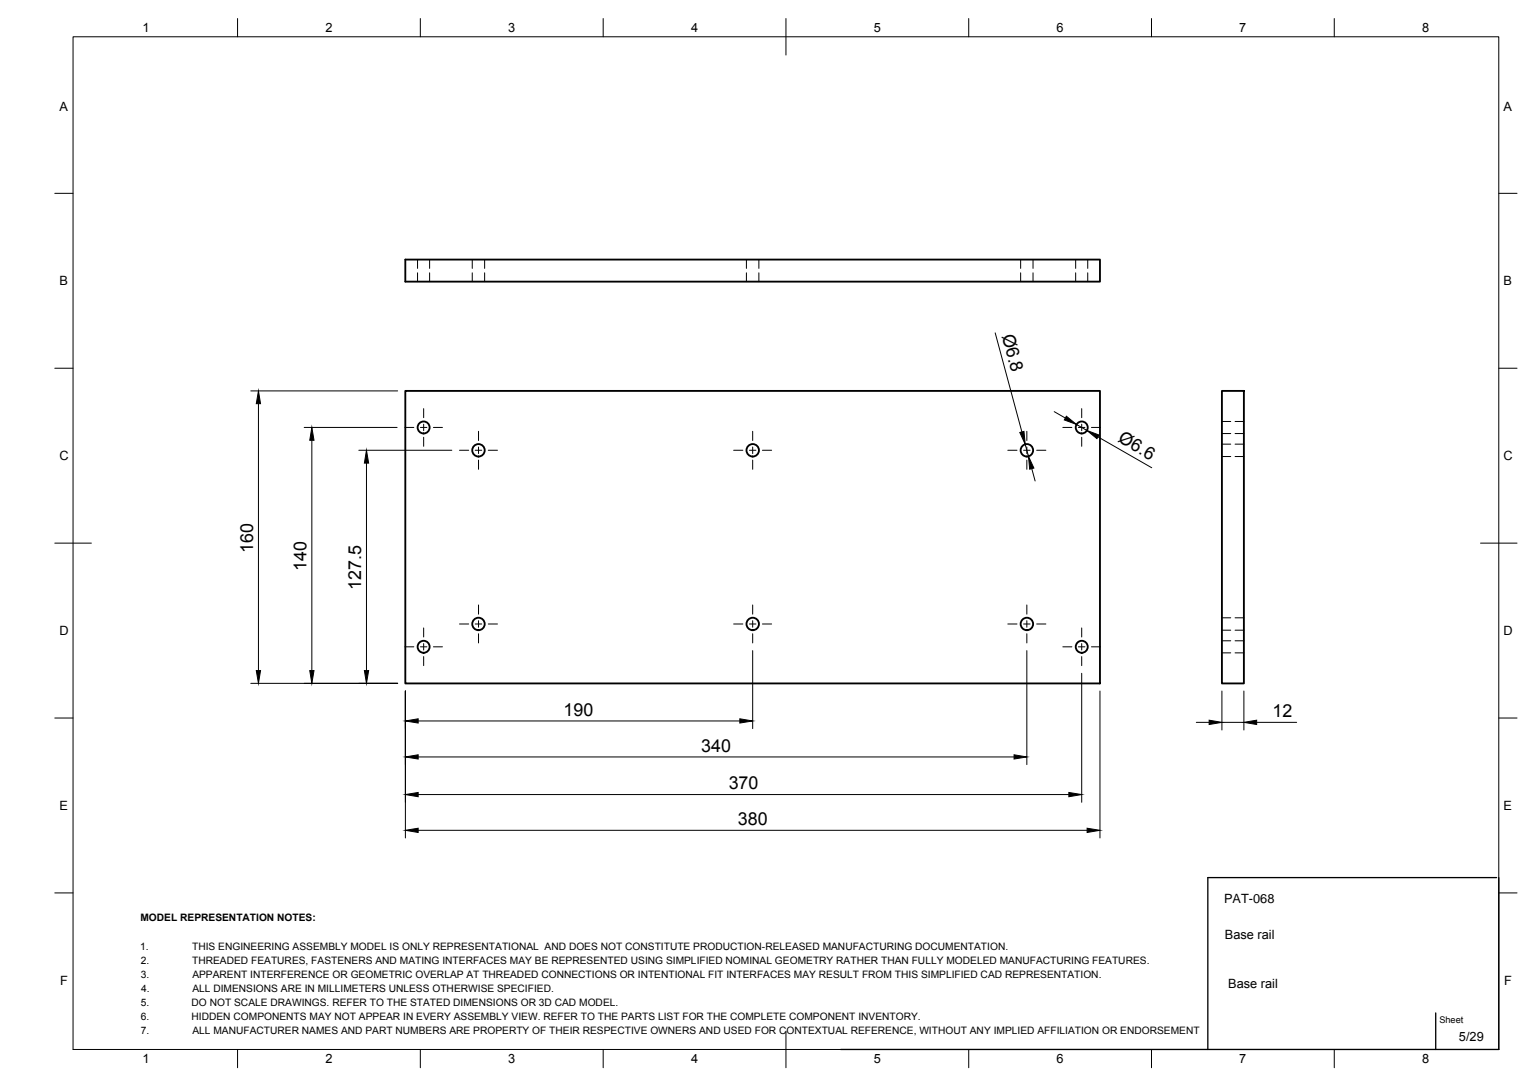
ISO-10303-21;
HEADER;
/* Generated by software containing ST-Developer
 * from STEP Tools, Inc. (www.steptools.com) 
 */

FILE_DESCRIPTION(
/* description */ ('Line shaft on three pillow blocks'),
/* implementation_level */ '2;1');

FILE_NAME(
/* name */ 'Base rail.step',
/* time_stamp */ '2026-10-27T10:49:19-07:00',
/* author */ (''),
/* organization */ (''),
/* preprocessor_version */ 'ST-DEVELOPER v20.2',
/* originating_system */ 'Autodesk Translation Framework v15.17.0.0',
/* authorisation */ '');

FILE_SCHEMA (('AUTOMOTIVE_DESIGN { 1 0 10303 214 3 1 1 }'));
ENDSEC;

DATA;
#10=MECHANICAL_DESIGN_GEOMETRIC_PRESENTATION_REPRESENTATION('',(#338),#8377);
#284=SHAPE_REPRESENTATION_RELATIONSHIP('SRR','None',#8499,#311);
#311=ADVANCED_BREP_SHAPE_REPRESENTATION('',(#366),#8348);
#338=STYLED_ITEM('',(#8697),#366);
#366=MANIFOLD_SOLID_BREP('Body1',#4324);
#391=FACE_BOUND('',#921,.T.);
#392=FACE_BOUND('',#922,.T.);
#393=FACE_BOUND('',#923,.T.);
#394=FACE_BOUND('',#924,.T.);
#395=FACE_BOUND('',#925,.T.);
#396=FACE_BOUND('',#926,.T.);
#397=FACE_BOUND('',#927,.T.);
#398=FACE_BOUND('',#928,.T.);
#399=FACE_BOUND('',#929,.T.);
#400=FACE_BOUND('',#930,.T.);
#401=FACE_BOUND('',#932,.T.);
#402=FACE_BOUND('',#933,.T.);
#403=FACE_BOUND('',#934,.T.);
#404=FACE_BOUND('',#935,.T.);
#405=FACE_BOUND('',#936,.T.);
#406=FACE_BOUND('',#937,.T.);
#407=FACE_BOUND('',#938,.T.);
#408=FACE_BOUND('',#939,.T.);
#409=FACE_BOUND('',#940,.T.);
#410=FACE_BOUND('',#941,.T.);
#488=PLANE('',#4686);
#489=PLANE('',#4687);
#490=PLANE('',#4688);
#491=PLANE('',#4689);
#492=PLANE('',#4690);
#493=PLANE('',#4691);
#654=FACE_OUTER_BOUND('',#906,.T.);
#655=FACE_OUTER_BOUND('',#907,.T.);
#656=FACE_OUTER_BOUND('',#908,.T.);
#657=FACE_OUTER_BOUND('',#909,.T.);
#658=FACE_OUTER_BOUND('',#910,.T.);
#659=FACE_OUTER_BOUND('',#911,.T.);
#660=FACE_OUTER_BOUND('',#912,.T.);
#661=FACE_OUTER_BOUND('',#913,.T.);
#662=FACE_OUTER_BOUND('',#914,.T.);
#663=FACE_OUTER_BOUND('',#915,.T.);
#664=FACE_OUTER_BOUND('',#916,.T.);
#665=FACE_OUTER_BOUND('',#917,.T.);
#666=FACE_OUTER_BOUND('',#918,.T.);
#667=FACE_OUTER_BOUND('',#919,.T.);
#668=FACE_OUTER_BOUND('',#920,.T.);
#669=FACE_OUTER_BOUND('',#931,.T.);
#906=EDGE_LOOP('',(#2949,#2950,#2951,#2952));
#907=EDGE_LOOP('',(#2953,#2954,#2955,#2956));
#908=EDGE_LOOP('',(#2957,#2958,#2959,#2960));
#909=EDGE_LOOP('',(#2961,#2962,#2963,#2964));
#910=EDGE_LOOP('',(#2965,#2966,#2967,#2968));
#911=EDGE_LOOP('',(#2969,#2970,#2971,#2972));
#912=EDGE_LOOP('',(#2973,#2974,#2975,#2976));
#913=EDGE_LOOP('',(#2977,#2978,#2979,#2980));
#914=EDGE_LOOP('',(#2981,#2982,#2983,#2984));
#915=EDGE_LOOP('',(#2985,#2986,#2987,#2988));
#916=EDGE_LOOP('',(#2989,#2990,#2991,#2992));
#917=EDGE_LOOP('',(#2993,#2994,#2995,#2996));
#918=EDGE_LOOP('',(#2997,#2998,#2999,#3000));
#919=EDGE_LOOP('',(#3001,#3002,#3003,#3004));
#920=EDGE_LOOP('',(#3005,#3006,#3007,#3008));
#921=EDGE_LOOP('',(#3009));
#922=EDGE_LOOP('',(#3010));
#923=EDGE_LOOP('',(#3011));
#924=EDGE_LOOP('',(#3012));
#925=EDGE_LOOP('',(#3013));
#926=EDGE_LOOP('',(#3014));
#927=EDGE_LOOP('',(#3015));
#928=EDGE_LOOP('',(#3016));
#929=EDGE_LOOP('',(#3017));
#930=EDGE_LOOP('',(#3018));
#931=EDGE_LOOP('',(#3019,#3020,#3021,#3022));
#932=EDGE_LOOP('',(#3023));
#933=EDGE_LOOP('',(#3024));
#934=EDGE_LOOP('',(#3025));
#935=EDGE_LOOP('',(#3026));
#936=EDGE_LOOP('',(#3027));
#937=EDGE_LOOP('',(#3028));
#938=EDGE_LOOP('',(#3029));
#939=EDGE_LOOP('',(#3030));
#940=EDGE_LOOP('',(#3031));
#941=EDGE_LOOP('',(#3032));
#1255=LINE('',#6472,#1582);
#1256=LINE('',#6478,#1583);
#1257=LINE('',#6484,#1584);
#1258=LINE('',#6490,#1585);
#1259=LINE('',#6496,#1586);
#1260=LINE('',#6502,#1587);
#1261=LINE('',#6508,#1588);
#1262=LINE('',#6514,#1589);
#1263=LINE('',#6520,#1590);
#1264=LINE('',#6526,#1591);
#1265=LINE('',#6531,#1592);
#1266=LINE('',#6533,#1593);
#1267=LINE('',#6535,#1594);
#1268=LINE('',#6536,#1595);
#1269=LINE('',#6539,#1596);
#1270=LINE('',#6541,#1597);
#1271=LINE('',#6542,#1598);
#1272=LINE('',#6545,#1599);
#1273=LINE('',#6547,#1600);
#1274=LINE('',#6548,#1601);
#1275=LINE('',#6550,#1602);
#1276=LINE('',#6551,#1603);
#1582=VECTOR('',#5158,0.33);
#1583=VECTOR('',#5165,0.33);
#1584=VECTOR('',#5172,0.33);
#1585=VECTOR('',#5179,0.33);
#1586=VECTOR('',#5186,0.34);
#1587=VECTOR('',#5193,0.34);
#1588=VECTOR('',#5200,0.34);
#1589=VECTOR('',#5207,0.34);
#1590=VECTOR('',#5214,0.34);
#1591=VECTOR('',#5221,0.34);
#1592=VECTOR('',#5226,1.);
#1593=VECTOR('',#5227,1.);
#1594=VECTOR('',#5228,1.);
#1595=VECTOR('',#5229,1.);
#1596=VECTOR('',#5232,1.);
#1597=VECTOR('',#5233,1.);
#1598=VECTOR('',#5234,1.);
#1599=VECTOR('',#5237,1.);
#1600=VECTOR('',#5238,1.);
#1601=VECTOR('',#5239,1.);
#1602=VECTOR('',#5242,1.);
#1603=VECTOR('',#5243,1.);
#1909=CIRCLE('',#4657,0.33);
#1910=CIRCLE('',#4658,0.33);
#1911=CIRCLE('',#4660,0.33);
#1912=CIRCLE('',#4661,0.33);
#1913=CIRCLE('',#4663,0.33);
#1914=CIRCLE('',#4664,0.33);
#1915=CIRCLE('',#4666,0.33);
#1916=CIRCLE('',#4667,0.33);
#1917=CIRCLE('',#4669,0.34);
#1918=CIRCLE('',#4670,0.34);
#1919=CIRCLE('',#4672,0.34);
#1920=CIRCLE('',#4673,0.34);
#1921=CIRCLE('',#4675,0.34);
#1922=CIRCLE('',#4676,0.34);
#1923=CIRCLE('',#4678,0.34);
#1924=CIRCLE('',#4679,0.34);
#1925=CIRCLE('',#4681,0.34);
#1926=CIRCLE('',#4682,0.34);
#1927=CIRCLE('',#4684,0.34);
#1928=CIRCLE('',#4685,0.34);
#2068=VERTEX_POINT('',#6469);
#2069=VERTEX_POINT('',#6471);
#2070=VERTEX_POINT('',#6475);
#2071=VERTEX_POINT('',#6477);
#2072=VERTEX_POINT('',#6481);
#2073=VERTEX_POINT('',#6483);
#2074=VERTEX_POINT('',#6487);
#2075=VERTEX_POINT('',#6489);
#2076=VERTEX_POINT('',#6493);
#2077=VERTEX_POINT('',#6495);
#2078=VERTEX_POINT('',#6499);
#2079=VERTEX_POINT('',#6501);
#2080=VERTEX_POINT('',#6505);
#2081=VERTEX_POINT('',#6507);
#2082=VERTEX_POINT('',#6511);
#2083=VERTEX_POINT('',#6513);
#2084=VERTEX_POINT('',#6517);
#2085=VERTEX_POINT('',#6519);
#2086=VERTEX_POINT('',#6523);
#2087=VERTEX_POINT('',#6525);
#2088=VERTEX_POINT('',#6529);
#2089=VERTEX_POINT('',#6530);
#2090=VERTEX_POINT('',#6532);
#2091=VERTEX_POINT('',#6534);
#2092=VERTEX_POINT('',#6538);
#2093=VERTEX_POINT('',#6540);
#2094=VERTEX_POINT('',#6544);
#2095=VERTEX_POINT('',#6546);
#2423=EDGE_CURVE('',#2068,#2068,#1909,.T.);
#2424=EDGE_CURVE('',#2068,#2069,#1255,.T.);
#2425=EDGE_CURVE('',#2069,#2069,#1910,.T.);
#2426=EDGE_CURVE('',#2070,#2070,#1911,.T.);
#2427=EDGE_CURVE('',#2070,#2071,#1256,.T.);
#2428=EDGE_CURVE('',#2071,#2071,#1912,.T.);
#2429=EDGE_CURVE('',#2072,#2072,#1913,.T.);
#2430=EDGE_CURVE('',#2072,#2073,#1257,.T.);
#2431=EDGE_CURVE('',#2073,#2073,#1914,.T.);
#2432=EDGE_CURVE('',#2074,#2074,#1915,.T.);
#2433=EDGE_CURVE('',#2074,#2075,#1258,.T.);
#2434=EDGE_CURVE('',#2075,#2075,#1916,.T.);
#2435=EDGE_CURVE('',#2076,#2076,#1917,.T.);
#2436=EDGE_CURVE('',#2076,#2077,#1259,.T.);
#2437=EDGE_CURVE('',#2077,#2077,#1918,.T.);
#2438=EDGE_CURVE('',#2078,#2078,#1919,.T.);
#2439=EDGE_CURVE('',#2078,#2079,#1260,.T.);
#2440=EDGE_CURVE('',#2079,#2079,#1920,.T.);
#2441=EDGE_CURVE('',#2080,#2080,#1921,.T.);
#2442=EDGE_CURVE('',#2080,#2081,#1261,.T.);
#2443=EDGE_CURVE('',#2081,#2081,#1922,.T.);
#2444=EDGE_CURVE('',#2082,#2082,#1923,.T.);
#2445=EDGE_CURVE('',#2082,#2083,#1262,.T.);
#2446=EDGE_CURVE('',#2083,#2083,#1924,.T.);
#2447=EDGE_CURVE('',#2084,#2084,#1925,.T.);
#2448=EDGE_CURVE('',#2084,#2085,#1263,.T.);
#2449=EDGE_CURVE('',#2085,#2085,#1926,.T.);
#2450=EDGE_CURVE('',#2086,#2086,#1927,.T.);
#2451=EDGE_CURVE('',#2086,#2087,#1264,.T.);
#2452=EDGE_CURVE('',#2087,#2087,#1928,.T.);
#2453=EDGE_CURVE('',#2088,#2089,#1265,.T.);
#2454=EDGE_CURVE('',#2089,#2090,#1266,.T.);
#2455=EDGE_CURVE('',#2091,#2090,#1267,.T.);
#2456=EDGE_CURVE('',#2088,#2091,#1268,.T.);
#2457=EDGE_CURVE('',#2092,#2088,#1269,.T.);
#2458=EDGE_CURVE('',#2093,#2091,#1270,.T.);
#2459=EDGE_CURVE('',#2092,#2093,#1271,.T.);
#2460=EDGE_CURVE('',#2094,#2092,#1272,.T.);
#2461=EDGE_CURVE('',#2095,#2093,#1273,.T.);
#2462=EDGE_CURVE('',#2094,#2095,#1274,.T.);
#2463=EDGE_CURVE('',#2089,#2094,#1275,.T.);
#2464=EDGE_CURVE('',#2090,#2095,#1276,.T.);
#2949=ORIENTED_EDGE('',*,*,#2423,.F.);
#2950=ORIENTED_EDGE('',*,*,#2424,.T.);
#2951=ORIENTED_EDGE('',*,*,#2425,.F.);
#2952=ORIENTED_EDGE('',*,*,#2424,.F.);
#2953=ORIENTED_EDGE('',*,*,#2426,.F.);
#2954=ORIENTED_EDGE('',*,*,#2427,.T.);
#2955=ORIENTED_EDGE('',*,*,#2428,.F.);
#2956=ORIENTED_EDGE('',*,*,#2427,.F.);
#2957=ORIENTED_EDGE('',*,*,#2429,.F.);
#2958=ORIENTED_EDGE('',*,*,#2430,.T.);
#2959=ORIENTED_EDGE('',*,*,#2431,.F.);
#2960=ORIENTED_EDGE('',*,*,#2430,.F.);
#2961=ORIENTED_EDGE('',*,*,#2432,.F.);
#2962=ORIENTED_EDGE('',*,*,#2433,.T.);
#2963=ORIENTED_EDGE('',*,*,#2434,.F.);
#2964=ORIENTED_EDGE('',*,*,#2433,.F.);
#2965=ORIENTED_EDGE('',*,*,#2435,.F.);
#2966=ORIENTED_EDGE('',*,*,#2436,.T.);
#2967=ORIENTED_EDGE('',*,*,#2437,.F.);
#2968=ORIENTED_EDGE('',*,*,#2436,.F.);
#2969=ORIENTED_EDGE('',*,*,#2438,.F.);
#2970=ORIENTED_EDGE('',*,*,#2439,.T.);
#2971=ORIENTED_EDGE('',*,*,#2440,.F.);
#2972=ORIENTED_EDGE('',*,*,#2439,.F.);
#2973=ORIENTED_EDGE('',*,*,#2441,.F.);
#2974=ORIENTED_EDGE('',*,*,#2442,.T.);
#2975=ORIENTED_EDGE('',*,*,#2443,.F.);
#2976=ORIENTED_EDGE('',*,*,#2442,.F.);
#2977=ORIENTED_EDGE('',*,*,#2444,.F.);
#2978=ORIENTED_EDGE('',*,*,#2445,.T.);
#2979=ORIENTED_EDGE('',*,*,#2446,.F.);
#2980=ORIENTED_EDGE('',*,*,#2445,.F.);
#2981=ORIENTED_EDGE('',*,*,#2447,.F.);
#2982=ORIENTED_EDGE('',*,*,#2448,.T.);
#2983=ORIENTED_EDGE('',*,*,#2449,.F.);
#2984=ORIENTED_EDGE('',*,*,#2448,.F.);
#2985=ORIENTED_EDGE('',*,*,#2450,.F.);
#2986=ORIENTED_EDGE('',*,*,#2451,.T.);
#2987=ORIENTED_EDGE('',*,*,#2452,.F.);
#2988=ORIENTED_EDGE('',*,*,#2451,.F.);
#2989=ORIENTED_EDGE('',*,*,#2453,.T.);
#2990=ORIENTED_EDGE('',*,*,#2454,.T.);
#2991=ORIENTED_EDGE('',*,*,#2455,.F.);
#2992=ORIENTED_EDGE('',*,*,#2456,.F.);
#2993=ORIENTED_EDGE('',*,*,#2457,.T.);
#2994=ORIENTED_EDGE('',*,*,#2456,.T.);
#2995=ORIENTED_EDGE('',*,*,#2458,.F.);
#2996=ORIENTED_EDGE('',*,*,#2459,.F.);
#2997=ORIENTED_EDGE('',*,*,#2460,.T.);
#2998=ORIENTED_EDGE('',*,*,#2459,.T.);
#2999=ORIENTED_EDGE('',*,*,#2461,.F.);
#3000=ORIENTED_EDGE('',*,*,#2462,.F.);
#3001=ORIENTED_EDGE('',*,*,#2463,.T.);
#3002=ORIENTED_EDGE('',*,*,#2462,.T.);
#3003=ORIENTED_EDGE('',*,*,#2464,.F.);
#3004=ORIENTED_EDGE('',*,*,#2454,.F.);
#3005=ORIENTED_EDGE('',*,*,#2464,.T.);
#3006=ORIENTED_EDGE('',*,*,#2461,.T.);
#3007=ORIENTED_EDGE('',*,*,#2458,.T.);
#3008=ORIENTED_EDGE('',*,*,#2455,.T.);
#3009=ORIENTED_EDGE('',*,*,#2437,.T.);
#3010=ORIENTED_EDGE('',*,*,#2440,.T.);
#3011=ORIENTED_EDGE('',*,*,#2443,.T.);
#3012=ORIENTED_EDGE('',*,*,#2446,.T.);
#3013=ORIENTED_EDGE('',*,*,#2449,.T.);
#3014=ORIENTED_EDGE('',*,*,#2452,.T.);
#3015=ORIENTED_EDGE('',*,*,#2434,.T.);
#3016=ORIENTED_EDGE('',*,*,#2431,.T.);
#3017=ORIENTED_EDGE('',*,*,#2428,.T.);
#3018=ORIENTED_EDGE('',*,*,#2425,.T.);
#3019=ORIENTED_EDGE('',*,*,#2463,.F.);
#3020=ORIENTED_EDGE('',*,*,#2453,.F.);
#3021=ORIENTED_EDGE('',*,*,#2457,.F.);
#3022=ORIENTED_EDGE('',*,*,#2460,.F.);
#3023=ORIENTED_EDGE('',*,*,#2435,.T.);
#3024=ORIENTED_EDGE('',*,*,#2438,.T.);
#3025=ORIENTED_EDGE('',*,*,#2441,.T.);
#3026=ORIENTED_EDGE('',*,*,#2444,.T.);
#3027=ORIENTED_EDGE('',*,*,#2447,.T.);
#3028=ORIENTED_EDGE('',*,*,#2450,.T.);
#3029=ORIENTED_EDGE('',*,*,#2432,.T.);
#3030=ORIENTED_EDGE('',*,*,#2429,.T.);
#3031=ORIENTED_EDGE('',*,*,#2426,.T.);
#3032=ORIENTED_EDGE('',*,*,#2423,.T.);
#4001=CYLINDRICAL_SURFACE('',#4656,0.33);
#4002=CYLINDRICAL_SURFACE('',#4659,0.33);
#4003=CYLINDRICAL_SURFACE('',#4662,0.33);
#4004=CYLINDRICAL_SURFACE('',#4665,0.33);
#4005=CYLINDRICAL_SURFACE('',#4668,0.34);
#4006=CYLINDRICAL_SURFACE('',#4671,0.34);
#4007=CYLINDRICAL_SURFACE('',#4674,0.34);
#4008=CYLINDRICAL_SURFACE('',#4677,0.34);
#4009=CYLINDRICAL_SURFACE('',#4680,0.34);
#4010=CYLINDRICAL_SURFACE('',#4683,0.34);
#4072=ADVANCED_FACE('',(#654),#4001,.F.);
#4073=ADVANCED_FACE('',(#655),#4002,.F.);
#4074=ADVANCED_FACE('',(#656),#4003,.F.);
#4075=ADVANCED_FACE('',(#657),#4004,.F.);
#4076=ADVANCED_FACE('',(#658),#4005,.F.);
#4077=ADVANCED_FACE('',(#659),#4006,.F.);
#4078=ADVANCED_FACE('',(#660),#4007,.F.);
#4079=ADVANCED_FACE('',(#661),#4008,.F.);
#4080=ADVANCED_FACE('',(#662),#4009,.F.);
#4081=ADVANCED_FACE('',(#663),#4010,.F.);
#4082=ADVANCED_FACE('',(#664),#488,.T.);
#4083=ADVANCED_FACE('',(#665),#489,.T.);
#4084=ADVANCED_FACE('',(#666),#490,.T.);
#4085=ADVANCED_FACE('',(#667),#491,.T.);
#4086=ADVANCED_FACE('',(#668,#391,#392,#393,#394,#395,#396,#397,#398,#399,
#400),#492,.T.);
#4087=ADVANCED_FACE('',(#669,#401,#402,#403,#404,#405,#406,#407,#408,#409,
#410),#493,.F.);
#4324=CLOSED_SHELL('',(#4072,#4073,#4074,#4075,#4076,#4077,#4078,#4079,
#4080,#4081,#4082,#4083,#4084,#4085,#4086,#4087));
#4655=AXIS2_PLACEMENT_3D('',#6467,#5152,#5153);
#4656=AXIS2_PLACEMENT_3D('',#6468,#5154,#5155);
#4657=AXIS2_PLACEMENT_3D('',#6470,#5156,#5157);
#4658=AXIS2_PLACEMENT_3D('',#6473,#5159,#5160);
#4659=AXIS2_PLACEMENT_3D('',#6474,#5161,#5162);
#4660=AXIS2_PLACEMENT_3D('',#6476,#5163,#5164);
#4661=AXIS2_PLACEMENT_3D('',#6479,#5166,#5167);
#4662=AXIS2_PLACEMENT_3D('',#6480,#5168,#5169);
#4663=AXIS2_PLACEMENT_3D('',#6482,#5170,#5171);
#4664=AXIS2_PLACEMENT_3D('',#6485,#5173,#5174);
#4665=AXIS2_PLACEMENT_3D('',#6486,#5175,#5176);
#4666=AXIS2_PLACEMENT_3D('',#6488,#5177,#5178);
#4667=AXIS2_PLACEMENT_3D('',#6491,#5180,#5181);
#4668=AXIS2_PLACEMENT_3D('',#6492,#5182,#5183);
#4669=AXIS2_PLACEMENT_3D('',#6494,#5184,#5185);
#4670=AXIS2_PLACEMENT_3D('',#6497,#5187,#5188);
#4671=AXIS2_PLACEMENT_3D('',#6498,#5189,#5190);
#4672=AXIS2_PLACEMENT_3D('',#6500,#5191,#5192);
#4673=AXIS2_PLACEMENT_3D('',#6503,#5194,#5195);
#4674=AXIS2_PLACEMENT_3D('',#6504,#5196,#5197);
#4675=AXIS2_PLACEMENT_3D('',#6506,#5198,#5199);
#4676=AXIS2_PLACEMENT_3D('',#6509,#5201,#5202);
#4677=AXIS2_PLACEMENT_3D('',#6510,#5203,#5204);
#4678=AXIS2_PLACEMENT_3D('',#6512,#5205,#5206);
#4679=AXIS2_PLACEMENT_3D('',#6515,#5208,#5209);
#4680=AXIS2_PLACEMENT_3D('',#6516,#5210,#5211);
#4681=AXIS2_PLACEMENT_3D('',#6518,#5212,#5213);
#4682=AXIS2_PLACEMENT_3D('',#6521,#5215,#5216);
#4683=AXIS2_PLACEMENT_3D('',#6522,#5217,#5218);
#4684=AXIS2_PLACEMENT_3D('',#6524,#5219,#5220);
#4685=AXIS2_PLACEMENT_3D('',#6527,#5222,#5223);
#4686=AXIS2_PLACEMENT_3D('',#6528,#5224,#5225);
#4687=AXIS2_PLACEMENT_3D('',#6537,#5230,#5231);
#4688=AXIS2_PLACEMENT_3D('',#6543,#5235,#5236);
#4689=AXIS2_PLACEMENT_3D('',#6549,#5240,#5241);
#4690=AXIS2_PLACEMENT_3D('',#6552,#5244,#5245);
#4691=AXIS2_PLACEMENT_3D('',#6553,#5246,#5247);
#5152=DIRECTION('axis',(0.,0.,1.));
#5153=DIRECTION('refdir',(1.,0.,0.));
#5154=DIRECTION('center_axis',(0.,0.,1.));
#5155=DIRECTION('ref_axis',(1.,0.,0.));
#5156=DIRECTION('center_axis',(0.,0.,1.));
#5157=DIRECTION('ref_axis',(1.,0.,0.));
#5158=DIRECTION('',(0.,0.,1.));
#5159=DIRECTION('center_axis',(0.,0.,-1.));
#5160=DIRECTION('ref_axis',(1.,0.,0.));
#5161=DIRECTION('center_axis',(0.,0.,1.));
#5162=DIRECTION('ref_axis',(1.,0.,0.));
#5163=DIRECTION('center_axis',(0.,0.,1.));
#5164=DIRECTION('ref_axis',(1.,0.,0.));
#5165=DIRECTION('',(0.,0.,1.));
#5166=DIRECTION('center_axis',(0.,0.,-1.));
#5167=DIRECTION('ref_axis',(1.,0.,0.));
#5168=DIRECTION('center_axis',(0.,0.,1.));
#5169=DIRECTION('ref_axis',(1.,0.,0.));
#5170=DIRECTION('center_axis',(0.,0.,1.));
#5171=DIRECTION('ref_axis',(1.,0.,0.));
#5172=DIRECTION('',(0.,0.,1.));
#5173=DIRECTION('center_axis',(0.,0.,-1.));
#5174=DIRECTION('ref_axis',(1.,0.,0.));
#5175=DIRECTION('center_axis',(0.,0.,1.));
#5176=DIRECTION('ref_axis',(1.,0.,0.));
#5177=DIRECTION('center_axis',(0.,0.,1.));
#5178=DIRECTION('ref_axis',(1.,0.,0.));
#5179=DIRECTION('',(0.,0.,1.));
#5180=DIRECTION('center_axis',(0.,0.,-1.));
#5181=DIRECTION('ref_axis',(1.,0.,0.));
#5182=DIRECTION('center_axis',(0.,0.,1.));
#5183=DIRECTION('ref_axis',(1.,0.,0.));
#5184=DIRECTION('center_axis',(0.,0.,1.));
#5185=DIRECTION('ref_axis',(1.,0.,0.));
#5186=DIRECTION('',(0.,0.,1.));
#5187=DIRECTION('center_axis',(0.,0.,-1.));
#5188=DIRECTION('ref_axis',(1.,0.,0.));
#5189=DIRECTION('center_axis',(0.,0.,1.));
#5190=DIRECTION('ref_axis',(1.,0.,0.));
#5191=DIRECTION('center_axis',(0.,0.,1.));
#5192=DIRECTION('ref_axis',(1.,0.,0.));
#5193=DIRECTION('',(0.,0.,1.));
#5194=DIRECTION('center_axis',(0.,0.,-1.));
#5195=DIRECTION('ref_axis',(1.,0.,0.));
#5196=DIRECTION('center_axis',(0.,0.,1.));
#5197=DIRECTION('ref_axis',(1.,0.,0.));
#5198=DIRECTION('center_axis',(0.,0.,1.));
#5199=DIRECTION('ref_axis',(1.,0.,0.));
#5200=DIRECTION('',(0.,0.,1.));
#5201=DIRECTION('center_axis',(0.,0.,-1.));
#5202=DIRECTION('ref_axis',(1.,0.,0.));
#5203=DIRECTION('center_axis',(0.,0.,1.));
#5204=DIRECTION('ref_axis',(1.,0.,0.));
#5205=DIRECTION('center_axis',(0.,0.,1.));
#5206=DIRECTION('ref_axis',(1.,0.,0.));
#5207=DIRECTION('',(0.,0.,1.));
#5208=DIRECTION('center_axis',(0.,0.,-1.));
#5209=DIRECTION('ref_axis',(1.,0.,0.));
#5210=DIRECTION('center_axis',(0.,0.,1.));
#5211=DIRECTION('ref_axis',(1.,0.,0.));
#5212=DIRECTION('center_axis',(0.,0.,1.));
#5213=DIRECTION('ref_axis',(1.,0.,0.));
#5214=DIRECTION('',(0.,0.,1.));
#5215=DIRECTION('center_axis',(0.,0.,-1.));
#5216=DIRECTION('ref_axis',(1.,0.,0.));
#5217=DIRECTION('center_axis',(0.,0.,1.));
#5218=DIRECTION('ref_axis',(1.,0.,0.));
#5219=DIRECTION('center_axis',(0.,0.,1.));
#5220=DIRECTION('ref_axis',(1.,0.,0.));
#5221=DIRECTION('',(0.,0.,1.));
#5222=DIRECTION('center_axis',(0.,0.,-1.));
#5223=DIRECTION('ref_axis',(1.,0.,0.));
#5224=DIRECTION('center_axis',(0.,1.,0.));
#5225=DIRECTION('ref_axis',(-1.,0.,0.));
#5226=DIRECTION('',(-1.,0.,0.));
#5227=DIRECTION('',(0.,0.,1.));
#5228=DIRECTION('',(-1.,0.,0.));
#5229=DIRECTION('',(0.,0.,1.));
#5230=DIRECTION('center_axis',(1.,0.,0.));
#5231=DIRECTION('ref_axis',(0.,1.,0.));
#5232=DIRECTION('',(0.,1.,0.));
#5233=DIRECTION('',(0.,1.,0.));
#5234=DIRECTION('',(0.,0.,1.));
#5235=DIRECTION('center_axis',(0.,-1.,0.));
#5236=DIRECTION('ref_axis',(1.,0.,0.));
#5237=DIRECTION('',(1.,0.,0.));
#5238=DIRECTION('',(1.,0.,0.));
#5239=DIRECTION('',(0.,0.,1.));
#5240=DIRECTION('center_axis',(-1.,0.,0.));
#5241=DIRECTION('ref_axis',(0.,-1.,0.));
#5242=DIRECTION('',(0.,-1.,0.));
#5243=DIRECTION('',(0.,-1.,0.));
#5244=DIRECTION('center_axis',(0.,0.,1.));
#5245=DIRECTION('ref_axis',(1.,0.,0.));
#5246=DIRECTION('center_axis',(0.,0.,1.));
#5247=DIRECTION('ref_axis',(1.,0.,0.));
#6467=CARTESIAN_POINT('',(0.,0.,0.));
#6468=CARTESIAN_POINT('Origin',(6.,-3.,-0.1));
#6469=CARTESIAN_POINT('',(5.67,-3.,0.));
#6470=CARTESIAN_POINT('Origin',(6.,-3.,0.));
#6471=CARTESIAN_POINT('',(5.67,-3.,1.2));
#6472=CARTESIAN_POINT('',(5.67,-3.,-0.1));
#6473=CARTESIAN_POINT('Origin',(6.,-3.,1.2));
#6474=CARTESIAN_POINT('Origin',(-6.,33.,-0.1));
#6475=CARTESIAN_POINT('',(-6.33,33.,0.));
#6476=CARTESIAN_POINT('Origin',(-6.,33.,0.));
#6477=CARTESIAN_POINT('',(-6.33,33.,1.2));
#6478=CARTESIAN_POINT('',(-6.33,33.,-0.1));
#6479=CARTESIAN_POINT('Origin',(-6.,33.,1.2));
#6480=CARTESIAN_POINT('Origin',(-6.,-3.,-0.1));
#6481=CARTESIAN_POINT('',(-6.33,-3.,0.));
#6482=CARTESIAN_POINT('Origin',(-6.,-3.,0.));
#6483=CARTESIAN_POINT('',(-6.33,-3.,1.2));
#6484=CARTESIAN_POINT('',(-6.33,-3.,-0.1));
#6485=CARTESIAN_POINT('Origin',(-6.,-3.,1.2));
#6486=CARTESIAN_POINT('Origin',(6.,33.,-0.1));
#6487=CARTESIAN_POINT('',(5.67,33.,0.));
#6488=CARTESIAN_POINT('Origin',(6.,33.,0.));
#6489=CARTESIAN_POINT('',(5.67,33.,1.2));
#6490=CARTESIAN_POINT('',(5.67,33.,-0.1));
#6491=CARTESIAN_POINT('Origin',(6.,33.,1.2));
#6492=CARTESIAN_POINT('Origin',(4.75,15.,-0.1));
#6493=CARTESIAN_POINT('',(4.41,15.,0.));
#6494=CARTESIAN_POINT('Origin',(4.75,15.,0.));
#6495=CARTESIAN_POINT('',(4.41,15.,1.2));
#6496=CARTESIAN_POINT('',(4.41,15.,-0.1));
#6497=CARTESIAN_POINT('Origin',(4.75,15.,1.2));
#6498=CARTESIAN_POINT('Origin',(-4.75,0.,-0.1));
#6499=CARTESIAN_POINT('',(-5.09,-4.163799117101E-17,0.));
#6500=CARTESIAN_POINT('Origin',(-4.75,0.,0.));
#6501=CARTESIAN_POINT('',(-5.09,4.163799117101E-17,1.2));
#6502=CARTESIAN_POINT('',(-5.09,-4.163799117101E-17,-0.1));
#6503=CARTESIAN_POINT('Origin',(-4.75,0.,1.2));
#6504=CARTESIAN_POINT('Origin',(-4.75,15.,-0.1));
#6505=CARTESIAN_POINT('',(-5.09,15.,0.));
#6506=CARTESIAN_POINT('Origin',(-4.75,15.,0.));
#6507=CARTESIAN_POINT('',(-5.09,15.,1.2));
#6508=CARTESIAN_POINT('',(-5.09,15.,-0.1));
#6509=CARTESIAN_POINT('Origin',(-4.75,15.,1.2));
#6510=CARTESIAN_POINT('Origin',(-4.75,30.,-0.1));
#6511=CARTESIAN_POINT('',(-5.09,30.,0.));
#6512=CARTESIAN_POINT('Origin',(-4.75,30.,0.));
#6513=CARTESIAN_POINT('',(-5.09,30.,1.2));
#6514=CARTESIAN_POINT('',(-5.09,30.,-0.1));
#6515=CARTESIAN_POINT('Origin',(-4.75,30.,1.2));
#6516=CARTESIAN_POINT('Origin',(4.75,0.,-0.1));
#6517=CARTESIAN_POINT('',(4.41,-4.163799117101E-17,0.));
#6518=CARTESIAN_POINT('Origin',(4.75,0.,0.));
#6519=CARTESIAN_POINT('',(4.41,4.163799117101E-17,1.2));
#6520=CARTESIAN_POINT('',(4.41,-4.163799117101E-17,-0.1));
#6521=CARTESIAN_POINT('Origin',(4.75,0.,1.2));
#6522=CARTESIAN_POINT('Origin',(4.75,30.,-0.1));
#6523=CARTESIAN_POINT('',(4.41,30.,0.));
#6524=CARTESIAN_POINT('Origin',(4.75,30.,0.));
#6525=CARTESIAN_POINT('',(4.41,30.,1.2));
#6526=CARTESIAN_POINT('',(4.41,30.,-0.1));
#6527=CARTESIAN_POINT('Origin',(4.75,30.,1.2));
#6528=CARTESIAN_POINT('Origin',(8.,34.,0.));
#6529=CARTESIAN_POINT('',(8.,34.,0.));
#6530=CARTESIAN_POINT('',(-8.,34.,0.));
#6531=CARTESIAN_POINT('',(8.,34.,0.));
#6532=CARTESIAN_POINT('',(-8.,34.,1.2));
#6533=CARTESIAN_POINT('',(-8.,34.,0.));
#6534=CARTESIAN_POINT('',(8.,34.,1.2));
#6535=CARTESIAN_POINT('',(8.,34.,1.2));
#6536=CARTESIAN_POINT('',(8.,34.,0.));
#6537=CARTESIAN_POINT('Origin',(8.,-4.,0.));
#6538=CARTESIAN_POINT('',(8.,-4.,0.));
#6539=CARTESIAN_POINT('',(8.,-4.,0.));
#6540=CARTESIAN_POINT('',(8.,-4.,1.2));
#6541=CARTESIAN_POINT('',(8.,-4.,1.2));
#6542=CARTESIAN_POINT('',(8.,-4.,0.));
#6543=CARTESIAN_POINT('Origin',(-8.,-4.,0.));
#6544=CARTESIAN_POINT('',(-8.,-4.,0.));
#6545=CARTESIAN_POINT('',(-8.,-4.,0.));
#6546=CARTESIAN_POINT('',(-8.,-4.,1.2));
#6547=CARTESIAN_POINT('',(-8.,-4.,1.2));
#6548=CARTESIAN_POINT('',(-8.,-4.,0.));
#6549=CARTESIAN_POINT('Origin',(-8.,34.,0.));
#6550=CARTESIAN_POINT('',(-8.,34.,0.));
#6551=CARTESIAN_POINT('',(-8.,34.,1.2));
#6552=CARTESIAN_POINT('Origin',(0.,15.,1.2));
#6553=CARTESIAN_POINT('Origin',(0.,15.,0.));
#8316=UNCERTAINTY_MEASURE_WITH_UNIT(LENGTH_MEASURE(0.001),#8378,
'DISTANCE_ACCURACY_VALUE',
'Maximum model space distance between geometric entities at asserted c
onnectivities');
#8345=UNCERTAINTY_MEASURE_WITH_UNIT(LENGTH_MEASURE(0.001),#8378,
'DISTANCE_ACCURACY_VALUE',
'Maximum model space distance between geometric entities at asserted c
onnectivities');
#8348=(
GEOMETRIC_REPRESENTATION_CONTEXT(3)
GLOBAL_UNCERTAINTY_ASSIGNED_CONTEXT((#8316))
GLOBAL_UNIT_ASSIGNED_CONTEXT((#8378,#8380,#8381))
REPRESENTATION_CONTEXT('','3D')
);
#8377=(
GEOMETRIC_REPRESENTATION_CONTEXT(3)
GLOBAL_UNCERTAINTY_ASSIGNED_CONTEXT((#8345))
GLOBAL_UNIT_ASSIGNED_CONTEXT((#8378,#8380,#8381))
REPRESENTATION_CONTEXT('','3D')
);
#8378=(
LENGTH_UNIT()
NAMED_UNIT(*)
SI_UNIT(.CENTI.,.METRE.)
);
#8380=(
NAMED_UNIT(*)
PLANE_ANGLE_UNIT()
SI_UNIT($,.RADIAN.)
);
#8381=(
NAMED_UNIT(*)
SI_UNIT($,.STERADIAN.)
SOLID_ANGLE_UNIT()
);
#8384=SHAPE_DEFINITION_REPRESENTATION(#8415,#8499);
#8415=PRODUCT_DEFINITION_SHAPE('',$,#8531);
#8499=SHAPE_REPRESENTATION('',(#4655),#8348);
#8528=PRODUCT_DEFINITION_CONTEXT('part definition',#8623,'design');
#8531=PRODUCT_DEFINITION('Base rail','Base rail',#8562,#8528);
#8562=PRODUCT_DEFINITION_FORMATION('',$,#8627);
#8623=APPLICATION_CONTEXT(
'Core Data for Automotive Mechanical Design Process');
#8624=PRODUCT_CONTEXT('part definition',#8623,'mechanical');
#8627=PRODUCT('Base rail','Base rail','Base rail',(#8624));
#8691=COLOUR_RGB('Dark Blue',0.08,0.2,0.34);
#8692=FILL_AREA_STYLE_COLOUR('',#8691);
#8693=FILL_AREA_STYLE('',(#8692));
#8694=SURFACE_STYLE_FILL_AREA(#8693);
#8695=SURFACE_SIDE_STYLE('',(#8694));
#8696=SURFACE_STYLE_USAGE(.BOTH.,#8695);
#8697=PRESENTATION_STYLE_ASSIGNMENT((#8696));
ENDSEC;
END-ISO-10303-21;
